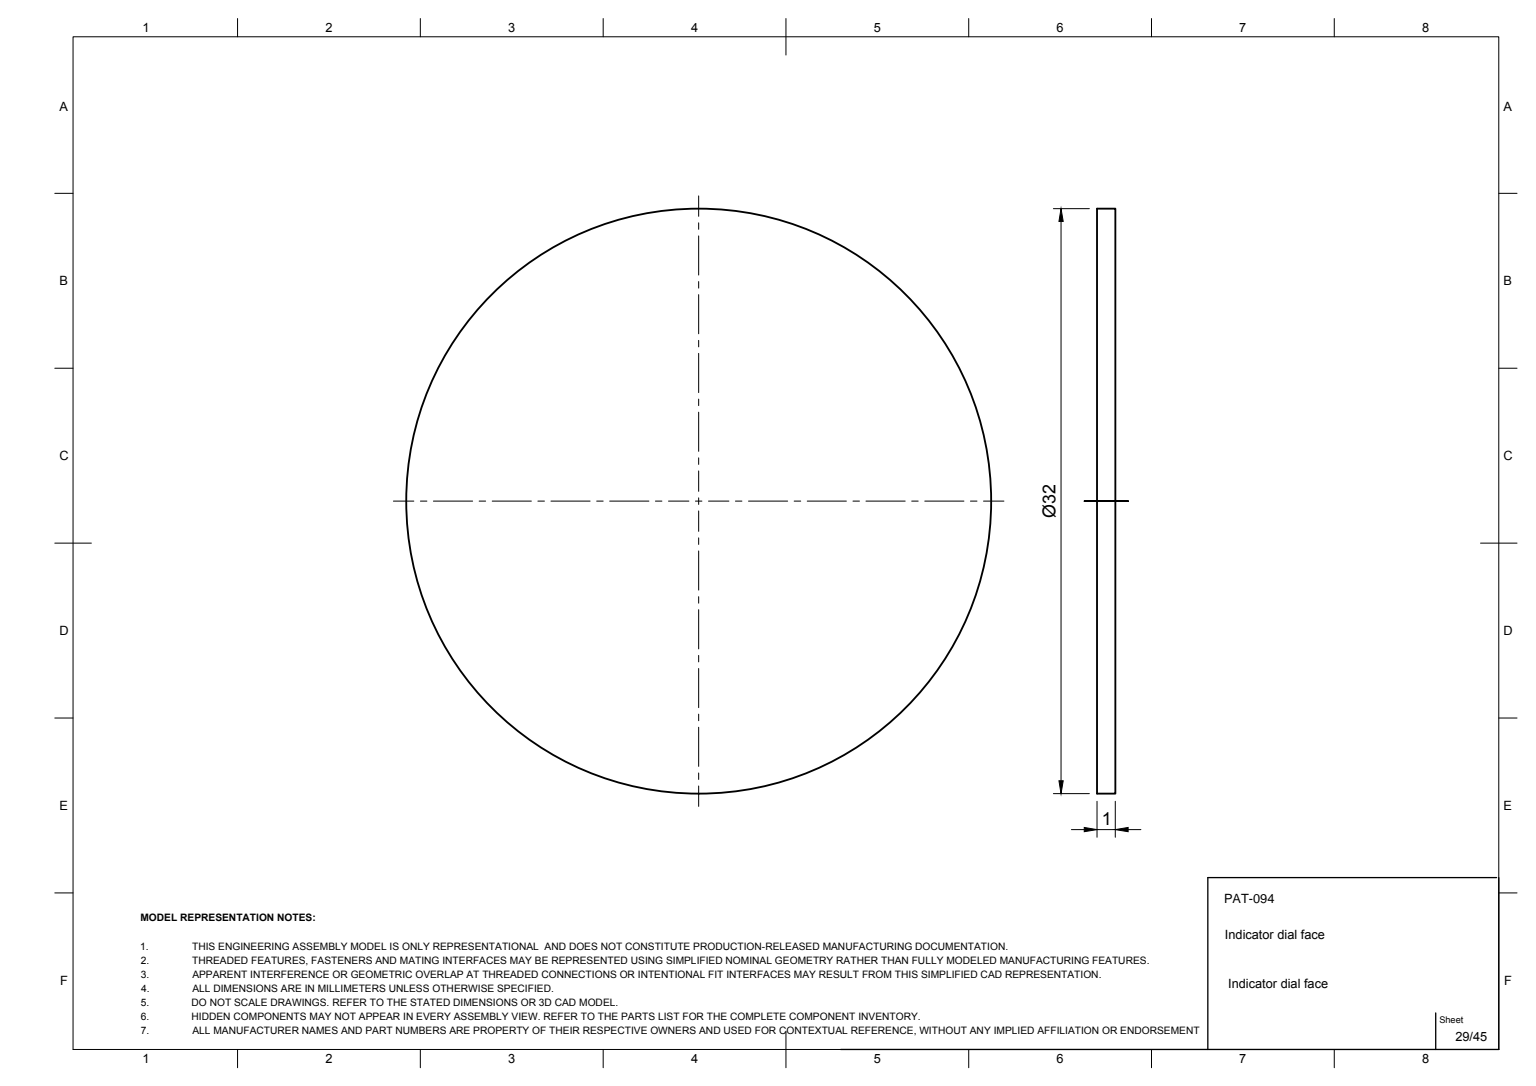
ISO-10303-21;
HEADER;
/* Generated by software containing ST-Developer
 * from STEP Tools, Inc. (www.steptools.com) 
 */

FILE_DESCRIPTION(
/* description */ ('Shaft runout checking stand'),
/* implementation_level */ '2;1');

FILE_NAME(
/* name */ 'Indicator dial face.step',
/* time_stamp */ '2026-11-02T21:12:33-08:00',
/* author */ (''),
/* organization */ (''),
/* preprocessor_version */ 'ST-DEVELOPER v20.2',
/* originating_system */ 'Autodesk Translation Framework v15.17.0.0',
/* authorisation */ '');

FILE_SCHEMA (('AUTOMOTIVE_DESIGN { 1 0 10303 214 3 1 1 }'));
ENDSEC;

DATA;
#10=MECHANICAL_DESIGN_GEOMETRIC_PRESENTATION_REPRESENTATION('',(#491),#11748);
#405=SHAPE_REPRESENTATION_RELATIONSHIP('SRR','None',#11954,#448);
#448=ADVANCED_BREP_SHAPE_REPRESENTATION('',(#539),#11730);
#491=STYLED_ITEM('',(#12169),#539);
#539=MANIFOLD_SOLID_BREP('Body1',#6237);
#836=CIRCLE('',#7210,1.6);
#837=CIRCLE('',#7211,1.6);
#1011=CYLINDRICAL_SURFACE('',#7209,1.6);
#1317=FACE_OUTER_BOUND('',#1775,.T.);
#1318=FACE_OUTER_BOUND('',#1776,.T.);
#1319=FACE_OUTER_BOUND('',#1777,.T.);
#1775=EDGE_LOOP('',(#5284,#5285,#5286,#5287));
#1776=EDGE_LOOP('',(#5288));
#1777=EDGE_LOOP('',(#5289));
#2312=LINE('',#10860,#2779);
#2779=VECTOR('',#8873,1.6);
#3214=VERTEX_POINT('',#10857);
#3215=VERTEX_POINT('',#10859);
#3928=EDGE_CURVE('',#3214,#3214,#836,.T.);
#3929=EDGE_CURVE('',#3214,#3215,#2312,.T.);
#3930=EDGE_CURVE('',#3215,#3215,#837,.T.);
#5284=ORIENTED_EDGE('',*,*,#3928,.F.);
#5285=ORIENTED_EDGE('',*,*,#3929,.T.);
#5286=ORIENTED_EDGE('',*,*,#3930,.T.);
#5287=ORIENTED_EDGE('',*,*,#3929,.F.);
#5288=ORIENTED_EDGE('',*,*,#3928,.T.);
#5289=ORIENTED_EDGE('',*,*,#3930,.F.);
#5798=PLANE('',#7212);
#5799=PLANE('',#7213);
#6117=ADVANCED_FACE('',(#1317),#1011,.T.);
#6118=ADVANCED_FACE('',(#1318),#5798,.T.);
#6119=ADVANCED_FACE('',(#1319),#5799,.F.);
#6237=CLOSED_SHELL('',(#6117,#6118,#6119));
#7208=AXIS2_PLACEMENT_3D('',#10855,#8867,#8868);
#7209=AXIS2_PLACEMENT_3D('',#10856,#8869,#8870);
#7210=AXIS2_PLACEMENT_3D('',#10858,#8871,#8872);
#7211=AXIS2_PLACEMENT_3D('',#10861,#8874,#8875);
#7212=AXIS2_PLACEMENT_3D('',#10862,#8876,#8877);
#7213=AXIS2_PLACEMENT_3D('',#10863,#8878,#8879);
#8867=DIRECTION('axis',(0.,0.,1.));
#8868=DIRECTION('refdir',(1.,0.,0.));
#8869=DIRECTION('center_axis',(0.,1.,0.));
#8870=DIRECTION('ref_axis',(1.,0.,0.));
#8871=DIRECTION('center_axis',(0.,1.,0.));
#8872=DIRECTION('ref_axis',(1.,0.,0.));
#8873=DIRECTION('',(0.,-1.,0.));
#8874=DIRECTION('center_axis',(0.,1.,0.));
#8875=DIRECTION('ref_axis',(1.,0.,0.));
#8876=DIRECTION('center_axis',(0.,1.,0.));
#8877=DIRECTION('ref_axis',(1.,0.,0.));
#8878=DIRECTION('center_axis',(0.,1.,0.));
#8879=DIRECTION('ref_axis',(1.,0.,0.));
#10855=CARTESIAN_POINT('',(0.,0.,0.));
#10856=CARTESIAN_POINT('Origin',(0.,0.6,15.2));
#10857=CARTESIAN_POINT('',(-1.6,0.7,15.2));
#10858=CARTESIAN_POINT('Origin',(0.,0.7,15.2));
#10859=CARTESIAN_POINT('',(-1.6,0.6,15.2));
#10860=CARTESIAN_POINT('',(-1.6,0.6,15.2));
#10861=CARTESIAN_POINT('Origin',(0.,0.6,15.2));
#10862=CARTESIAN_POINT('Origin',(0.,0.7,15.2));
#10863=CARTESIAN_POINT('Origin',(0.,0.6,15.2));
#11681=UNCERTAINTY_MEASURE_WITH_UNIT(LENGTH_MEASURE(0.001),#11749,
'DISTANCE_ACCURACY_VALUE',
'Maximum model space distance between geometric entities at asserted c
onnectivities');
#11699=UNCERTAINTY_MEASURE_WITH_UNIT(LENGTH_MEASURE(0.001),#11749,
'DISTANCE_ACCURACY_VALUE',
'Maximum model space distance between geometric entities at asserted c
onnectivities');
#11730=(
GEOMETRIC_REPRESENTATION_CONTEXT(3)
GLOBAL_UNCERTAINTY_ASSIGNED_CONTEXT((#11681))
GLOBAL_UNIT_ASSIGNED_CONTEXT((#11749,#11751,#11752))
REPRESENTATION_CONTEXT('','3D')
);
#11748=(
GEOMETRIC_REPRESENTATION_CONTEXT(3)
GLOBAL_UNCERTAINTY_ASSIGNED_CONTEXT((#11699))
GLOBAL_UNIT_ASSIGNED_CONTEXT((#11749,#11751,#11752))
REPRESENTATION_CONTEXT('','3D')
);
#11749=(
LENGTH_UNIT()
NAMED_UNIT(*)
SI_UNIT(.CENTI.,.METRE.)
);
#11751=(
NAMED_UNIT(*)
PLANE_ANGLE_UNIT()
SI_UNIT($,.RADIAN.)
);
#11752=(
NAMED_UNIT(*)
SI_UNIT($,.STERADIAN.)
SOLID_ANGLE_UNIT()
);
#11783=SHAPE_DEFINITION_REPRESENTATION(#11831,#11954);
#11831=PRODUCT_DEFINITION_SHAPE('',$,#12003);
#11954=SHAPE_REPRESENTATION('',(#7208),#11730);
#11972=PRODUCT_DEFINITION_CONTEXT('part definition',#12118,'design');
#12003=PRODUCT_DEFINITION('Indicator dial face','Indicator dial face',#12051,
#11972);
#12051=PRODUCT_DEFINITION_FORMATION('',$,#12150);
#12118=APPLICATION_CONTEXT(
'Core Data for Automotive Mechanical Design Process');
#12119=PRODUCT_CONTEXT('part definition',#12118,'mechanical');
#12150=PRODUCT('Indicator dial face','Indicator dial face',
'Indicator dial face',(#12119));
#12169=PRESENTATION_STYLE_ASSIGNMENT((#12174));
#12174=SURFACE_STYLE_USAGE(.BOTH.,#12179);
#12179=SURFACE_SIDE_STYLE('',(#12184));
#12184=SURFACE_STYLE_FILL_AREA(#12189);
#12189=FILL_AREA_STYLE('CAD Library Painted - Engineering blue',(#12194));
#12194=FILL_AREA_STYLE_COLOUR('CAD Library Painted - Engineering blue',
#12199);
#12199=COLOUR_RGB('CAD Library Painted - Engineering blue',0.12156862745098,
0.356862745098039,0.6);
ENDSEC;
END-ISO-10303-21;
